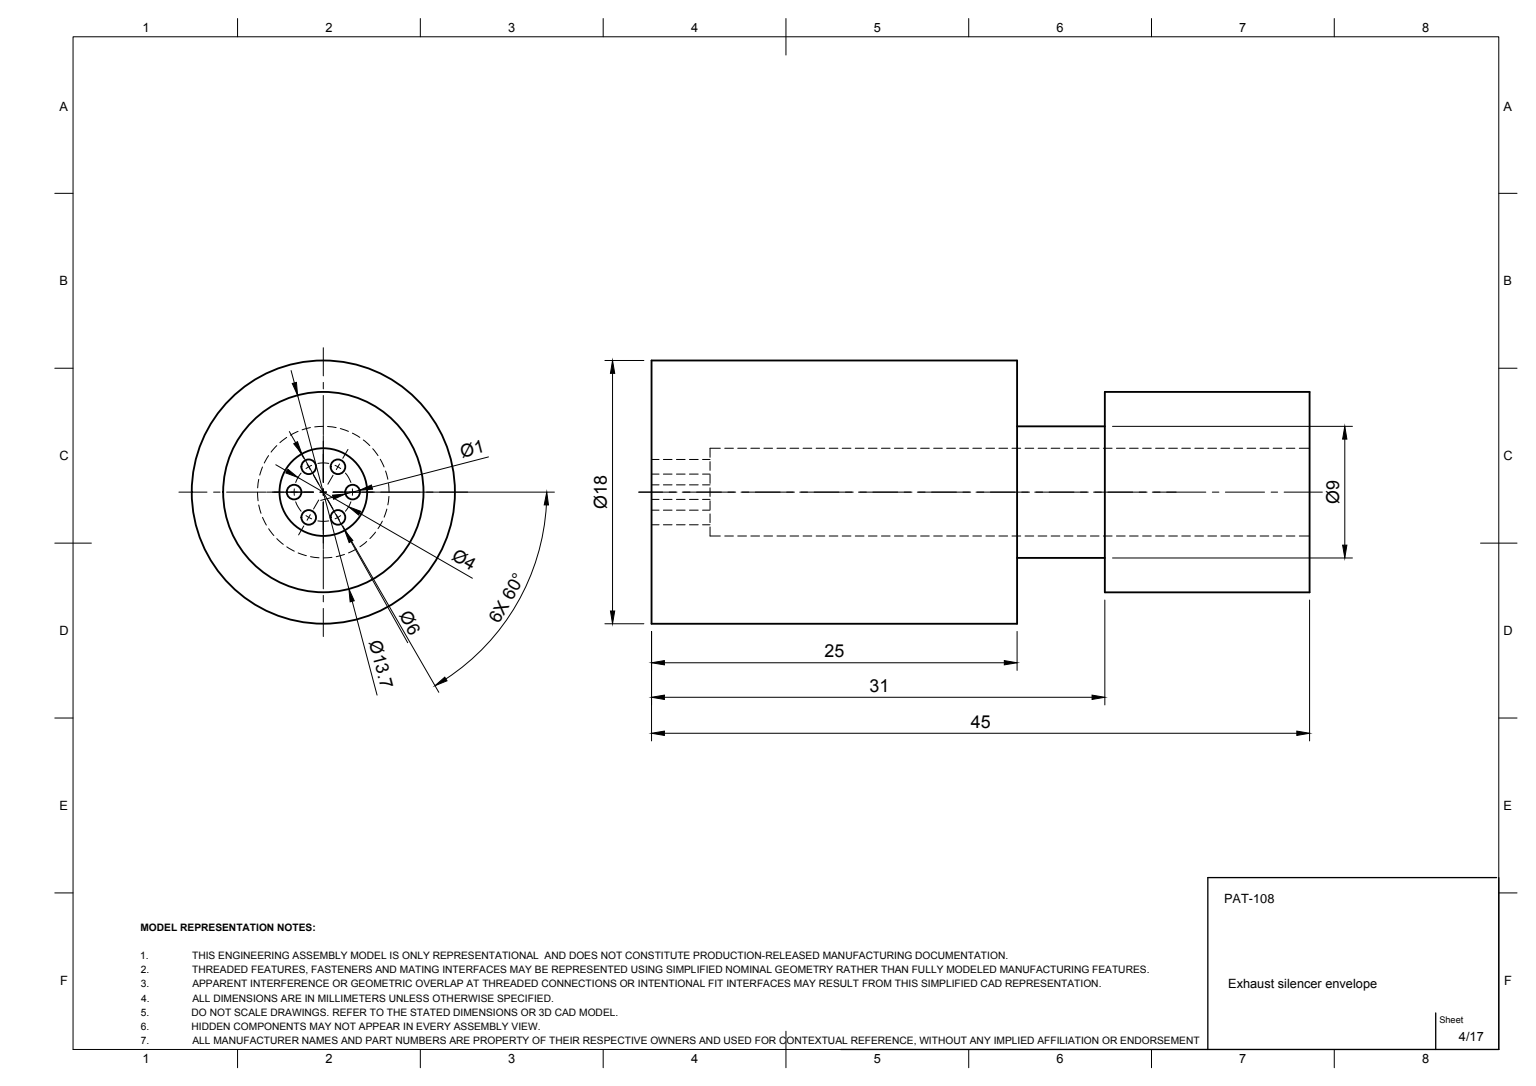
ISO-10303-21;
HEADER;
/* Generated by software containing ST-Developer
 * from STEP Tools, Inc. (www.steptools.com) 
 */

FILE_DESCRIPTION(
/* description */ ('Sub-base valve envelopes and connections'),
/* implementation_level */ '2;1');

FILE_NAME(
/* name */ 'Exhaust silencer envelope.step',
/* time_stamp */ '2026-10-29T15:55:44-07:00',
/* author */ (''),
/* organization */ (''),
/* preprocessor_version */ 'ST-DEVELOPER v20.2',
/* originating_system */ 'Autodesk Translation Framework v15.17.0.0',
/* authorisation */ '');

FILE_SCHEMA (('AUTOMOTIVE_DESIGN { 1 0 10303 214 3 1 1 }'));
ENDSEC;

DATA;
#10=MECHANICAL_DESIGN_GEOMETRIC_PRESENTATION_REPRESENTATION('',(#120),#6113);
#96=SHAPE_REPRESENTATION_RELATIONSHIP('SRR','None',#6169,#108);
#108=ADVANCED_BREP_SHAPE_REPRESENTATION('',(#132),#6100);
#120=STYLED_ITEM('',(#6329),#132);
#132=MANIFOLD_SOLID_BREP('Body1',#3359);
#176=FACE_BOUND('',#673,.T.);
#177=FACE_BOUND('',#674,.T.);
#178=FACE_BOUND('',#675,.T.);
#179=FACE_BOUND('',#676,.T.);
#180=FACE_BOUND('',#677,.T.);
#181=FACE_BOUND('',#678,.T.);
#182=FACE_BOUND('',#680,.T.);
#183=FACE_BOUND('',#683,.T.);
#184=FACE_BOUND('',#684,.T.);
#185=FACE_BOUND('',#685,.T.);
#186=FACE_BOUND('',#686,.T.);
#187=FACE_BOUND('',#687,.T.);
#188=FACE_BOUND('',#688,.T.);
#189=FACE_BOUND('',#693,.T.);
#190=FACE_BOUND('',#695,.T.);
#297=PLANE('',#3620);
#298=PLANE('',#3622);
#299=PLANE('',#3627);
#300=PLANE('',#3635);
#301=PLANE('',#3636);
#433=FACE_OUTER_BOUND('',#666,.T.);
#434=FACE_OUTER_BOUND('',#667,.T.);
#435=FACE_OUTER_BOUND('',#668,.T.);
#436=FACE_OUTER_BOUND('',#669,.T.);
#437=FACE_OUTER_BOUND('',#670,.T.);
#438=FACE_OUTER_BOUND('',#671,.T.);
#439=FACE_OUTER_BOUND('',#672,.T.);
#440=FACE_OUTER_BOUND('',#679,.T.);
#441=FACE_OUTER_BOUND('',#681,.T.);
#442=FACE_OUTER_BOUND('',#682,.T.);
#443=FACE_OUTER_BOUND('',#689,.T.);
#444=FACE_OUTER_BOUND('',#690,.T.);
#445=FACE_OUTER_BOUND('',#691,.T.);
#446=FACE_OUTER_BOUND('',#692,.T.);
#447=FACE_OUTER_BOUND('',#694,.T.);
#666=EDGE_LOOP('',(#2457,#2458,#2459,#2460));
#667=EDGE_LOOP('',(#2461,#2462,#2463,#2464));
#668=EDGE_LOOP('',(#2465,#2466,#2467,#2468));
#669=EDGE_LOOP('',(#2469,#2470,#2471,#2472));
#670=EDGE_LOOP('',(#2473,#2474,#2475,#2476));
#671=EDGE_LOOP('',(#2477,#2478,#2479,#2480));
#672=EDGE_LOOP('',(#2481));
#673=EDGE_LOOP('',(#2482));
#674=EDGE_LOOP('',(#2483));
#675=EDGE_LOOP('',(#2484));
#676=EDGE_LOOP('',(#2485));
#677=EDGE_LOOP('',(#2486));
#678=EDGE_LOOP('',(#2487));
#679=EDGE_LOOP('',(#2488));
#680=EDGE_LOOP('',(#2489));
#681=EDGE_LOOP('',(#2490,#2491,#2492,#2493));
#682=EDGE_LOOP('',(#2494));
#683=EDGE_LOOP('',(#2495));
#684=EDGE_LOOP('',(#2496));
#685=EDGE_LOOP('',(#2497));
#686=EDGE_LOOP('',(#2498));
#687=EDGE_LOOP('',(#2499));
#688=EDGE_LOOP('',(#2500));
#689=EDGE_LOOP('',(#2501,#2502,#2503,#2504));
#690=EDGE_LOOP('',(#2505,#2506,#2507,#2508));
#691=EDGE_LOOP('',(#2509,#2510,#2511,#2512));
#692=EDGE_LOOP('',(#2513));
#693=EDGE_LOOP('',(#2514));
#694=EDGE_LOOP('',(#2515));
#695=EDGE_LOOP('',(#2516));
#946=LINE('',#5390,#1180);
#947=LINE('',#5396,#1181);
#948=LINE('',#5402,#1182);
#949=LINE('',#5408,#1183);
#950=LINE('',#5414,#1184);
#951=LINE('',#5420,#1185);
#952=LINE('',#5433,#1186);
#953=LINE('',#5437,#1187);
#954=LINE('',#5441,#1188);
#955=LINE('',#5447,#1189);
#1180=VECTOR('',#4150,0.05);
#1181=VECTOR('',#4157,0.05);
#1182=VECTOR('',#4164,0.05);
#1183=VECTOR('',#4171,0.05);
#1184=VECTOR('',#4178,0.05);
#1185=VECTOR('',#4185,0.05);
#1186=VECTOR('',#4202,0.9);
#1187=VECTOR('',#4207,0.45);
#1188=VECTOR('',#4212,0.3);
#1189=VECTOR('',#4219,0.685);
#1417=CIRCLE('',#3603,0.05);
#1418=CIRCLE('',#3604,0.05);
#1419=CIRCLE('',#3606,0.05);
#1420=CIRCLE('',#3607,0.05);
#1421=CIRCLE('',#3609,0.05);
#1422=CIRCLE('',#3610,0.05);
#1423=CIRCLE('',#3612,0.05);
#1424=CIRCLE('',#3613,0.05);
#1425=CIRCLE('',#3615,0.05);
#1426=CIRCLE('',#3616,0.05);
#1427=CIRCLE('',#3618,0.05);
#1428=CIRCLE('',#3619,0.05);
#1429=CIRCLE('',#3621,0.3);
#1430=CIRCLE('',#3623,0.9);
#1431=CIRCLE('',#3624,0.45);
#1432=CIRCLE('',#3626,0.9);
#1433=CIRCLE('',#3629,0.45);
#1434=CIRCLE('',#3631,0.3);
#1435=CIRCLE('',#3633,0.685);
#1436=CIRCLE('',#3634,0.685);
#1611=VERTEX_POINT('',#5387);
#1612=VERTEX_POINT('',#5389);
#1613=VERTEX_POINT('',#5393);
#1614=VERTEX_POINT('',#5395);
#1615=VERTEX_POINT('',#5399);
#1616=VERTEX_POINT('',#5401);
#1617=VERTEX_POINT('',#5405);
#1618=VERTEX_POINT('',#5407);
#1619=VERTEX_POINT('',#5411);
#1620=VERTEX_POINT('',#5413);
#1621=VERTEX_POINT('',#5417);
#1622=VERTEX_POINT('',#5419);
#1623=VERTEX_POINT('',#5423);
#1624=VERTEX_POINT('',#5426);
#1625=VERTEX_POINT('',#5428);
#1626=VERTEX_POINT('',#5431);
#1627=VERTEX_POINT('',#5436);
#1628=VERTEX_POINT('',#5440);
#1629=VERTEX_POINT('',#5444);
#1630=VERTEX_POINT('',#5446);
#1926=EDGE_CURVE('',#1611,#1611,#1417,.T.);
#1927=EDGE_CURVE('',#1611,#1612,#946,.T.);
#1928=EDGE_CURVE('',#1612,#1612,#1418,.T.);
#1929=EDGE_CURVE('',#1613,#1613,#1419,.T.);
#1930=EDGE_CURVE('',#1613,#1614,#947,.T.);
#1931=EDGE_CURVE('',#1614,#1614,#1420,.T.);
#1932=EDGE_CURVE('',#1615,#1615,#1421,.T.);
#1933=EDGE_CURVE('',#1615,#1616,#948,.T.);
#1934=EDGE_CURVE('',#1616,#1616,#1422,.T.);
#1935=EDGE_CURVE('',#1617,#1617,#1423,.T.);
#1936=EDGE_CURVE('',#1617,#1618,#949,.T.);
#1937=EDGE_CURVE('',#1618,#1618,#1424,.T.);
#1938=EDGE_CURVE('',#1619,#1619,#1425,.T.);
#1939=EDGE_CURVE('',#1619,#1620,#950,.T.);
#1940=EDGE_CURVE('',#1620,#1620,#1426,.T.);
#1941=EDGE_CURVE('',#1621,#1621,#1427,.T.);
#1942=EDGE_CURVE('',#1621,#1622,#951,.T.);
#1943=EDGE_CURVE('',#1622,#1622,#1428,.T.);
#1944=EDGE_CURVE('',#1623,#1623,#1429,.T.);
#1945=EDGE_CURVE('',#1624,#1624,#1430,.T.);
#1946=EDGE_CURVE('',#1625,#1625,#1431,.T.);
#1947=EDGE_CURVE('',#1626,#1626,#1432,.T.);
#1948=EDGE_CURVE('',#1626,#1624,#952,.T.);
#1949=EDGE_CURVE('',#1625,#1627,#953,.T.);
#1950=EDGE_CURVE('',#1627,#1627,#1433,.T.);
#1951=EDGE_CURVE('',#1623,#1628,#954,.T.);
#1952=EDGE_CURVE('',#1628,#1628,#1434,.T.);
#1953=EDGE_CURVE('',#1629,#1629,#1435,.T.);
#1954=EDGE_CURVE('',#1629,#1630,#955,.T.);
#1955=EDGE_CURVE('',#1630,#1630,#1436,.T.);
#2457=ORIENTED_EDGE('',*,*,#1926,.F.);
#2458=ORIENTED_EDGE('',*,*,#1927,.T.);
#2459=ORIENTED_EDGE('',*,*,#1928,.F.);
#2460=ORIENTED_EDGE('',*,*,#1927,.F.);
#2461=ORIENTED_EDGE('',*,*,#1929,.F.);
#2462=ORIENTED_EDGE('',*,*,#1930,.T.);
#2463=ORIENTED_EDGE('',*,*,#1931,.F.);
#2464=ORIENTED_EDGE('',*,*,#1930,.F.);
#2465=ORIENTED_EDGE('',*,*,#1932,.F.);
#2466=ORIENTED_EDGE('',*,*,#1933,.T.);
#2467=ORIENTED_EDGE('',*,*,#1934,.F.);
#2468=ORIENTED_EDGE('',*,*,#1933,.F.);
#2469=ORIENTED_EDGE('',*,*,#1935,.F.);
#2470=ORIENTED_EDGE('',*,*,#1936,.T.);
#2471=ORIENTED_EDGE('',*,*,#1937,.F.);
#2472=ORIENTED_EDGE('',*,*,#1936,.F.);
#2473=ORIENTED_EDGE('',*,*,#1938,.F.);
#2474=ORIENTED_EDGE('',*,*,#1939,.T.);
#2475=ORIENTED_EDGE('',*,*,#1940,.F.);
#2476=ORIENTED_EDGE('',*,*,#1939,.F.);
#2477=ORIENTED_EDGE('',*,*,#1941,.F.);
#2478=ORIENTED_EDGE('',*,*,#1942,.T.);
#2479=ORIENTED_EDGE('',*,*,#1943,.F.);
#2480=ORIENTED_EDGE('',*,*,#1942,.F.);
#2481=ORIENTED_EDGE('',*,*,#1944,.F.);
#2482=ORIENTED_EDGE('',*,*,#1941,.T.);
#2483=ORIENTED_EDGE('',*,*,#1938,.T.);
#2484=ORIENTED_EDGE('',*,*,#1935,.T.);
#2485=ORIENTED_EDGE('',*,*,#1932,.T.);
#2486=ORIENTED_EDGE('',*,*,#1929,.T.);
#2487=ORIENTED_EDGE('',*,*,#1926,.T.);
#2488=ORIENTED_EDGE('',*,*,#1945,.F.);
#2489=ORIENTED_EDGE('',*,*,#1946,.F.);
#2490=ORIENTED_EDGE('',*,*,#1947,.F.);
#2491=ORIENTED_EDGE('',*,*,#1948,.T.);
#2492=ORIENTED_EDGE('',*,*,#1945,.T.);
#2493=ORIENTED_EDGE('',*,*,#1948,.F.);
#2494=ORIENTED_EDGE('',*,*,#1947,.T.);
#2495=ORIENTED_EDGE('',*,*,#1943,.T.);
#2496=ORIENTED_EDGE('',*,*,#1940,.T.);
#2497=ORIENTED_EDGE('',*,*,#1937,.T.);
#2498=ORIENTED_EDGE('',*,*,#1934,.T.);
#2499=ORIENTED_EDGE('',*,*,#1931,.T.);
#2500=ORIENTED_EDGE('',*,*,#1928,.T.);
#2501=ORIENTED_EDGE('',*,*,#1946,.T.);
#2502=ORIENTED_EDGE('',*,*,#1949,.T.);
#2503=ORIENTED_EDGE('',*,*,#1950,.F.);
#2504=ORIENTED_EDGE('',*,*,#1949,.F.);
#2505=ORIENTED_EDGE('',*,*,#1944,.T.);
#2506=ORIENTED_EDGE('',*,*,#1951,.T.);
#2507=ORIENTED_EDGE('',*,*,#1952,.T.);
#2508=ORIENTED_EDGE('',*,*,#1951,.F.);
#2509=ORIENTED_EDGE('',*,*,#1953,.F.);
#2510=ORIENTED_EDGE('',*,*,#1954,.T.);
#2511=ORIENTED_EDGE('',*,*,#1955,.T.);
#2512=ORIENTED_EDGE('',*,*,#1954,.F.);
#2513=ORIENTED_EDGE('',*,*,#1953,.T.);
#2514=ORIENTED_EDGE('',*,*,#1950,.T.);
#2515=ORIENTED_EDGE('',*,*,#1955,.F.);
#2516=ORIENTED_EDGE('',*,*,#1952,.F.);
#3102=CYLINDRICAL_SURFACE('',#3602,0.05);
#3103=CYLINDRICAL_SURFACE('',#3605,0.05);
#3104=CYLINDRICAL_SURFACE('',#3608,0.05);
#3105=CYLINDRICAL_SURFACE('',#3611,0.05);
#3106=CYLINDRICAL_SURFACE('',#3614,0.05);
#3107=CYLINDRICAL_SURFACE('',#3617,0.05);
#3108=CYLINDRICAL_SURFACE('',#3625,0.9);
#3109=CYLINDRICAL_SURFACE('',#3628,0.45);
#3110=CYLINDRICAL_SURFACE('',#3630,0.3);
#3111=CYLINDRICAL_SURFACE('',#3632,0.685);
#3206=ADVANCED_FACE('',(#433),#3102,.F.);
#3207=ADVANCED_FACE('',(#434),#3103,.F.);
#3208=ADVANCED_FACE('',(#435),#3104,.F.);
#3209=ADVANCED_FACE('',(#436),#3105,.F.);
#3210=ADVANCED_FACE('',(#437),#3106,.F.);
#3211=ADVANCED_FACE('',(#438),#3107,.F.);
#3212=ADVANCED_FACE('',(#439,#176,#177,#178,#179,#180,#181),#297,.F.);
#3213=ADVANCED_FACE('',(#440,#182),#298,.F.);
#3214=ADVANCED_FACE('',(#441),#3108,.T.);
#3215=ADVANCED_FACE('',(#442,#183,#184,#185,#186,#187,#188),#299,.T.);
#3216=ADVANCED_FACE('',(#443),#3109,.T.);
#3217=ADVANCED_FACE('',(#444),#3110,.F.);
#3218=ADVANCED_FACE('',(#445),#3111,.T.);
#3219=ADVANCED_FACE('',(#446,#189),#300,.T.);
#3220=ADVANCED_FACE('',(#447,#190),#301,.F.);
#3359=CLOSED_SHELL('',(#3206,#3207,#3208,#3209,#3210,#3211,#3212,#3213,
#3214,#3215,#3216,#3217,#3218,#3219,#3220));
#3601=AXIS2_PLACEMENT_3D('',#5385,#4144,#4145);
#3602=AXIS2_PLACEMENT_3D('',#5386,#4146,#4147);
#3603=AXIS2_PLACEMENT_3D('',#5388,#4148,#4149);
#3604=AXIS2_PLACEMENT_3D('',#5391,#4151,#4152);
#3605=AXIS2_PLACEMENT_3D('',#5392,#4153,#4154);
#3606=AXIS2_PLACEMENT_3D('',#5394,#4155,#4156);
#3607=AXIS2_PLACEMENT_3D('',#5397,#4158,#4159);
#3608=AXIS2_PLACEMENT_3D('',#5398,#4160,#4161);
#3609=AXIS2_PLACEMENT_3D('',#5400,#4162,#4163);
#3610=AXIS2_PLACEMENT_3D('',#5403,#4165,#4166);
#3611=AXIS2_PLACEMENT_3D('',#5404,#4167,#4168);
#3612=AXIS2_PLACEMENT_3D('',#5406,#4169,#4170);
#3613=AXIS2_PLACEMENT_3D('',#5409,#4172,#4173);
#3614=AXIS2_PLACEMENT_3D('',#5410,#4174,#4175);
#3615=AXIS2_PLACEMENT_3D('',#5412,#4176,#4177);
#3616=AXIS2_PLACEMENT_3D('',#5415,#4179,#4180);
#3617=AXIS2_PLACEMENT_3D('',#5416,#4181,#4182);
#3618=AXIS2_PLACEMENT_3D('',#5418,#4183,#4184);
#3619=AXIS2_PLACEMENT_3D('',#5421,#4186,#4187);
#3620=AXIS2_PLACEMENT_3D('',#5422,#4188,#4189);
#3621=AXIS2_PLACEMENT_3D('',#5424,#4190,#4191);
#3622=AXIS2_PLACEMENT_3D('',#5425,#4192,#4193);
#3623=AXIS2_PLACEMENT_3D('',#5427,#4194,#4195);
#3624=AXIS2_PLACEMENT_3D('',#5429,#4196,#4197);
#3625=AXIS2_PLACEMENT_3D('',#5430,#4198,#4199);
#3626=AXIS2_PLACEMENT_3D('',#5432,#4200,#4201);
#3627=AXIS2_PLACEMENT_3D('',#5434,#4203,#4204);
#3628=AXIS2_PLACEMENT_3D('',#5435,#4205,#4206);
#3629=AXIS2_PLACEMENT_3D('',#5438,#4208,#4209);
#3630=AXIS2_PLACEMENT_3D('',#5439,#4210,#4211);
#3631=AXIS2_PLACEMENT_3D('',#5442,#4213,#4214);
#3632=AXIS2_PLACEMENT_3D('',#5443,#4215,#4216);
#3633=AXIS2_PLACEMENT_3D('',#5445,#4217,#4218);
#3634=AXIS2_PLACEMENT_3D('',#5448,#4220,#4221);
#3635=AXIS2_PLACEMENT_3D('',#5449,#4222,#4223);
#3636=AXIS2_PLACEMENT_3D('',#5450,#4224,#4225);
#4144=DIRECTION('axis',(0.,0.,1.));
#4145=DIRECTION('refdir',(1.,0.,0.));
#4146=DIRECTION('center_axis',(1.,0.,0.));
#4147=DIRECTION('ref_axis',(0.,0.,-1.));
#4148=DIRECTION('center_axis',(1.,0.,0.));
#4149=DIRECTION('ref_axis',(0.,0.,-1.));
#4150=DIRECTION('',(1.,0.,0.));
#4151=DIRECTION('center_axis',(-1.,0.,0.));
#4152=DIRECTION('ref_axis',(0.,0.,-1.));
#4153=DIRECTION('center_axis',(1.,0.,0.));
#4154=DIRECTION('ref_axis',(0.,0.,-1.));
#4155=DIRECTION('center_axis',(1.,0.,0.));
#4156=DIRECTION('ref_axis',(0.,0.,-1.));
#4157=DIRECTION('',(1.,0.,0.));
#4158=DIRECTION('center_axis',(-1.,0.,0.));
#4159=DIRECTION('ref_axis',(0.,0.,-1.));
#4160=DIRECTION('center_axis',(1.,0.,0.));
#4161=DIRECTION('ref_axis',(0.,0.,-1.));
#4162=DIRECTION('center_axis',(1.,0.,0.));
#4163=DIRECTION('ref_axis',(0.,0.,-1.));
#4164=DIRECTION('',(1.,0.,0.));
#4165=DIRECTION('center_axis',(-1.,0.,0.));
#4166=DIRECTION('ref_axis',(0.,0.,-1.));
#4167=DIRECTION('center_axis',(1.,0.,0.));
#4168=DIRECTION('ref_axis',(0.,0.,-1.));
#4169=DIRECTION('center_axis',(1.,0.,0.));
#4170=DIRECTION('ref_axis',(0.,0.,-1.));
#4171=DIRECTION('',(1.,0.,0.));
#4172=DIRECTION('center_axis',(-1.,0.,0.));
#4173=DIRECTION('ref_axis',(0.,0.,-1.));
#4174=DIRECTION('center_axis',(1.,0.,0.));
#4175=DIRECTION('ref_axis',(0.,0.,-1.));
#4176=DIRECTION('center_axis',(1.,0.,0.));
#4177=DIRECTION('ref_axis',(0.,0.,-1.));
#4178=DIRECTION('',(1.,0.,0.));
#4179=DIRECTION('center_axis',(-1.,0.,0.));
#4180=DIRECTION('ref_axis',(0.,0.,-1.));
#4181=DIRECTION('center_axis',(1.,0.,0.));
#4182=DIRECTION('ref_axis',(0.,0.,-1.));
#4183=DIRECTION('center_axis',(1.,0.,0.));
#4184=DIRECTION('ref_axis',(0.,0.,-1.));
#4185=DIRECTION('',(1.,0.,0.));
#4186=DIRECTION('center_axis',(-1.,0.,0.));
#4187=DIRECTION('ref_axis',(0.,0.,-1.));
#4188=DIRECTION('center_axis',(1.,0.,0.));
#4189=DIRECTION('ref_axis',(0.,0.,-1.));
#4190=DIRECTION('center_axis',(1.,0.,0.));
#4191=DIRECTION('ref_axis',(0.,0.,-1.));
#4192=DIRECTION('center_axis',(1.,0.,0.));
#4193=DIRECTION('ref_axis',(0.,0.,-1.));
#4194=DIRECTION('center_axis',(1.,0.,0.));
#4195=DIRECTION('ref_axis',(0.,0.,-1.));
#4196=DIRECTION('center_axis',(-1.,0.,0.));
#4197=DIRECTION('ref_axis',(0.,0.,-1.));
#4198=DIRECTION('center_axis',(1.,0.,0.));
#4199=DIRECTION('ref_axis',(0.,0.,-1.));
#4200=DIRECTION('center_axis',(1.,0.,0.));
#4201=DIRECTION('ref_axis',(0.,0.,-1.));
#4202=DIRECTION('',(-1.,0.,0.));
#4203=DIRECTION('center_axis',(1.,0.,0.));
#4204=DIRECTION('ref_axis',(0.,0.,-1.));
#4205=DIRECTION('center_axis',(1.,0.,0.));
#4206=DIRECTION('ref_axis',(0.,0.,-1.));
#4207=DIRECTION('',(-1.,0.,0.));
#4208=DIRECTION('center_axis',(-1.,0.,0.));
#4209=DIRECTION('ref_axis',(0.,0.,-1.));
#4210=DIRECTION('center_axis',(1.,0.,0.));
#4211=DIRECTION('ref_axis',(0.,0.,-1.));
#4212=DIRECTION('',(-1.,0.,0.));
#4213=DIRECTION('center_axis',(-1.,0.,0.));
#4214=DIRECTION('ref_axis',(0.,0.,-1.));
#4215=DIRECTION('center_axis',(1.,0.,0.));
#4216=DIRECTION('ref_axis',(0.,0.,-1.));
#4217=DIRECTION('center_axis',(1.,0.,0.));
#4218=DIRECTION('ref_axis',(0.,0.,-1.));
#4219=DIRECTION('',(-1.,0.,0.));
#4220=DIRECTION('center_axis',(1.,0.,0.));
#4221=DIRECTION('ref_axis',(0.,0.,-1.));
#4222=DIRECTION('center_axis',(1.,0.,0.));
#4223=DIRECTION('ref_axis',(0.,0.,-1.));
#4224=DIRECTION('center_axis',(1.,0.,0.));
#4225=DIRECTION('ref_axis',(0.,0.,-1.));
#5385=CARTESIAN_POINT('',(0.,0.,0.));
#5386=CARTESIAN_POINT('Origin',(10.6,-1.6,0.826794919243112));
#5387=CARTESIAN_POINT('',(10.7,-1.6,0.876794919243112));
#5388=CARTESIAN_POINT('Origin',(10.7,-1.6,0.826794919243112));
#5389=CARTESIAN_POINT('',(11.1,-1.6,0.876794919243112));
#5390=CARTESIAN_POINT('',(10.6,-1.6,0.876794919243112));
#5391=CARTESIAN_POINT('Origin',(11.1,-1.6,0.826794919243112));
#5392=CARTESIAN_POINT('Origin',(10.6,-1.3,1.));
#5393=CARTESIAN_POINT('',(10.7,-1.3,1.05));
#5394=CARTESIAN_POINT('Origin',(10.7,-1.3,1.));
#5395=CARTESIAN_POINT('',(11.1,-1.3,1.05));
#5396=CARTESIAN_POINT('',(10.6,-1.3,1.05));
#5397=CARTESIAN_POINT('Origin',(11.1,-1.3,1.));
#5398=CARTESIAN_POINT('Origin',(10.6,-1.4,1.17320508075689));
#5399=CARTESIAN_POINT('',(10.7,-1.4,1.22320508075689));
#5400=CARTESIAN_POINT('Origin',(10.7,-1.4,1.17320508075689));
#5401=CARTESIAN_POINT('',(11.1,-1.4,1.22320508075689));
#5402=CARTESIAN_POINT('',(10.6,-1.4,1.22320508075689));
#5403=CARTESIAN_POINT('Origin',(11.1,-1.4,1.17320508075689));
#5404=CARTESIAN_POINT('Origin',(10.6,-1.6,1.17320508075689));
#5405=CARTESIAN_POINT('',(10.7,-1.6,1.22320508075689));
#5406=CARTESIAN_POINT('Origin',(10.7,-1.6,1.17320508075689));
#5407=CARTESIAN_POINT('',(11.1,-1.6,1.22320508075689));
#5408=CARTESIAN_POINT('',(10.6,-1.6,1.22320508075689));
#5409=CARTESIAN_POINT('Origin',(11.1,-1.6,1.17320508075689));
#5410=CARTESIAN_POINT('Origin',(10.6,-1.7,1.));
#5411=CARTESIAN_POINT('',(10.7,-1.7,1.05));
#5412=CARTESIAN_POINT('Origin',(10.7,-1.7,1.));
#5413=CARTESIAN_POINT('',(11.1,-1.7,1.05));
#5414=CARTESIAN_POINT('',(10.6,-1.7,1.05));
#5415=CARTESIAN_POINT('Origin',(11.1,-1.7,1.));
#5416=CARTESIAN_POINT('Origin',(10.6,-1.4,0.826794919243112));
#5417=CARTESIAN_POINT('',(10.7,-1.4,0.876794919243112));
#5418=CARTESIAN_POINT('Origin',(10.7,-1.4,0.826794919243112));
#5419=CARTESIAN_POINT('',(11.1,-1.4,0.876794919243112));
#5420=CARTESIAN_POINT('',(10.6,-1.4,0.876794919243112));
#5421=CARTESIAN_POINT('Origin',(11.1,-1.4,0.826794919243112));
#5422=CARTESIAN_POINT('Origin',(10.7,-1.5,1.));
#5423=CARTESIAN_POINT('',(10.7,-1.5,1.3));
#5424=CARTESIAN_POINT('Origin',(10.7,-1.5,1.));
#5425=CARTESIAN_POINT('Origin',(8.6,-1.5,1.));
#5426=CARTESIAN_POINT('',(8.6,-1.5,1.9));
#5427=CARTESIAN_POINT('Origin',(8.6,-1.5,1.));
#5428=CARTESIAN_POINT('',(8.6,-1.5,1.45));
#5429=CARTESIAN_POINT('Origin',(8.6,-1.5,1.));
#5430=CARTESIAN_POINT('Origin',(8.6,-1.5,1.));
#5431=CARTESIAN_POINT('',(11.1,-1.5,1.9));
#5432=CARTESIAN_POINT('Origin',(11.1,-1.5,1.));
#5433=CARTESIAN_POINT('',(8.6,-1.5,1.9));
#5434=CARTESIAN_POINT('Origin',(11.1,-1.5,1.));
#5435=CARTESIAN_POINT('Origin',(8.,-1.5,1.));
#5436=CARTESIAN_POINT('',(8.,-1.5,1.45));
#5437=CARTESIAN_POINT('',(8.,-1.5,1.45));
#5438=CARTESIAN_POINT('Origin',(8.,-1.5,1.));
#5439=CARTESIAN_POINT('Origin',(6.6,-1.5,1.));
#5440=CARTESIAN_POINT('',(6.6,-1.5,1.3));
#5441=CARTESIAN_POINT('',(6.6,-1.5,1.3));
#5442=CARTESIAN_POINT('Origin',(6.6,-1.5,1.));
#5443=CARTESIAN_POINT('Origin',(6.6,-1.5,1.));
#5444=CARTESIAN_POINT('',(8.,-1.5,1.685));
#5445=CARTESIAN_POINT('Origin',(8.,-1.5,1.));
#5446=CARTESIAN_POINT('',(6.6,-1.5,1.685));
#5447=CARTESIAN_POINT('',(6.6,-1.5,1.685));
#5448=CARTESIAN_POINT('Origin',(6.6,-1.5,1.));
#5449=CARTESIAN_POINT('Origin',(8.,-1.5,1.));
#5450=CARTESIAN_POINT('Origin',(6.6,-1.5,1.));
#6084=UNCERTAINTY_MEASURE_WITH_UNIT(LENGTH_MEASURE(0.001),#6114,
'DISTANCE_ACCURACY_VALUE',
'Maximum model space distance between geometric entities at asserted c
onnectivities');
#6097=UNCERTAINTY_MEASURE_WITH_UNIT(LENGTH_MEASURE(0.001),#6114,
'DISTANCE_ACCURACY_VALUE',
'Maximum model space distance between geometric entities at asserted c
onnectivities');
#6100=(
GEOMETRIC_REPRESENTATION_CONTEXT(3)
GLOBAL_UNCERTAINTY_ASSIGNED_CONTEXT((#6084))
GLOBAL_UNIT_ASSIGNED_CONTEXT((#6114,#6116,#6117))
REPRESENTATION_CONTEXT('','3D')
);
#6113=(
GEOMETRIC_REPRESENTATION_CONTEXT(3)
GLOBAL_UNCERTAINTY_ASSIGNED_CONTEXT((#6097))
GLOBAL_UNIT_ASSIGNED_CONTEXT((#6114,#6116,#6117))
REPRESENTATION_CONTEXT('','3D')
);
#6114=(
LENGTH_UNIT()
NAMED_UNIT(*)
SI_UNIT(.CENTI.,.METRE.)
);
#6116=(
NAMED_UNIT(*)
PLANE_ANGLE_UNIT()
SI_UNIT($,.RADIAN.)
);
#6117=(
NAMED_UNIT(*)
SI_UNIT($,.STERADIAN.)
SOLID_ANGLE_UNIT()
);
#6120=SHAPE_DEFINITION_REPRESENTATION(#6135,#6169);
#6135=PRODUCT_DEFINITION_SHAPE('',$,#6185);
#6169=SHAPE_REPRESENTATION('',(#3601),#6100);
#6182=PRODUCT_DEFINITION_CONTEXT('part definition',#6229,'design');
#6185=PRODUCT_DEFINITION('Exhaust silencer envelope',
'Exhaust silencer envelope',#6200,#6182);
#6200=PRODUCT_DEFINITION_FORMATION('',$,#6233);
#6229=APPLICATION_CONTEXT(
'Core Data for Automotive Mechanical Design Process');
#6230=PRODUCT_CONTEXT('part definition',#6229,'mechanical');
#6233=PRODUCT('Exhaust silencer envelope','Exhaust silencer envelope',
'Exhaust silencer envelope',(#6230));
#6323=COLOUR_RGB('Off White',0.89,0.88,0.83);
#6324=FILL_AREA_STYLE_COLOUR('',#6323);
#6325=FILL_AREA_STYLE('',(#6324));
#6326=SURFACE_STYLE_FILL_AREA(#6325);
#6327=SURFACE_SIDE_STYLE('',(#6326));
#6328=SURFACE_STYLE_USAGE(.BOTH.,#6327);
#6329=PRESENTATION_STYLE_ASSIGNMENT((#6328));
ENDSEC;
END-ISO-10303-21;
